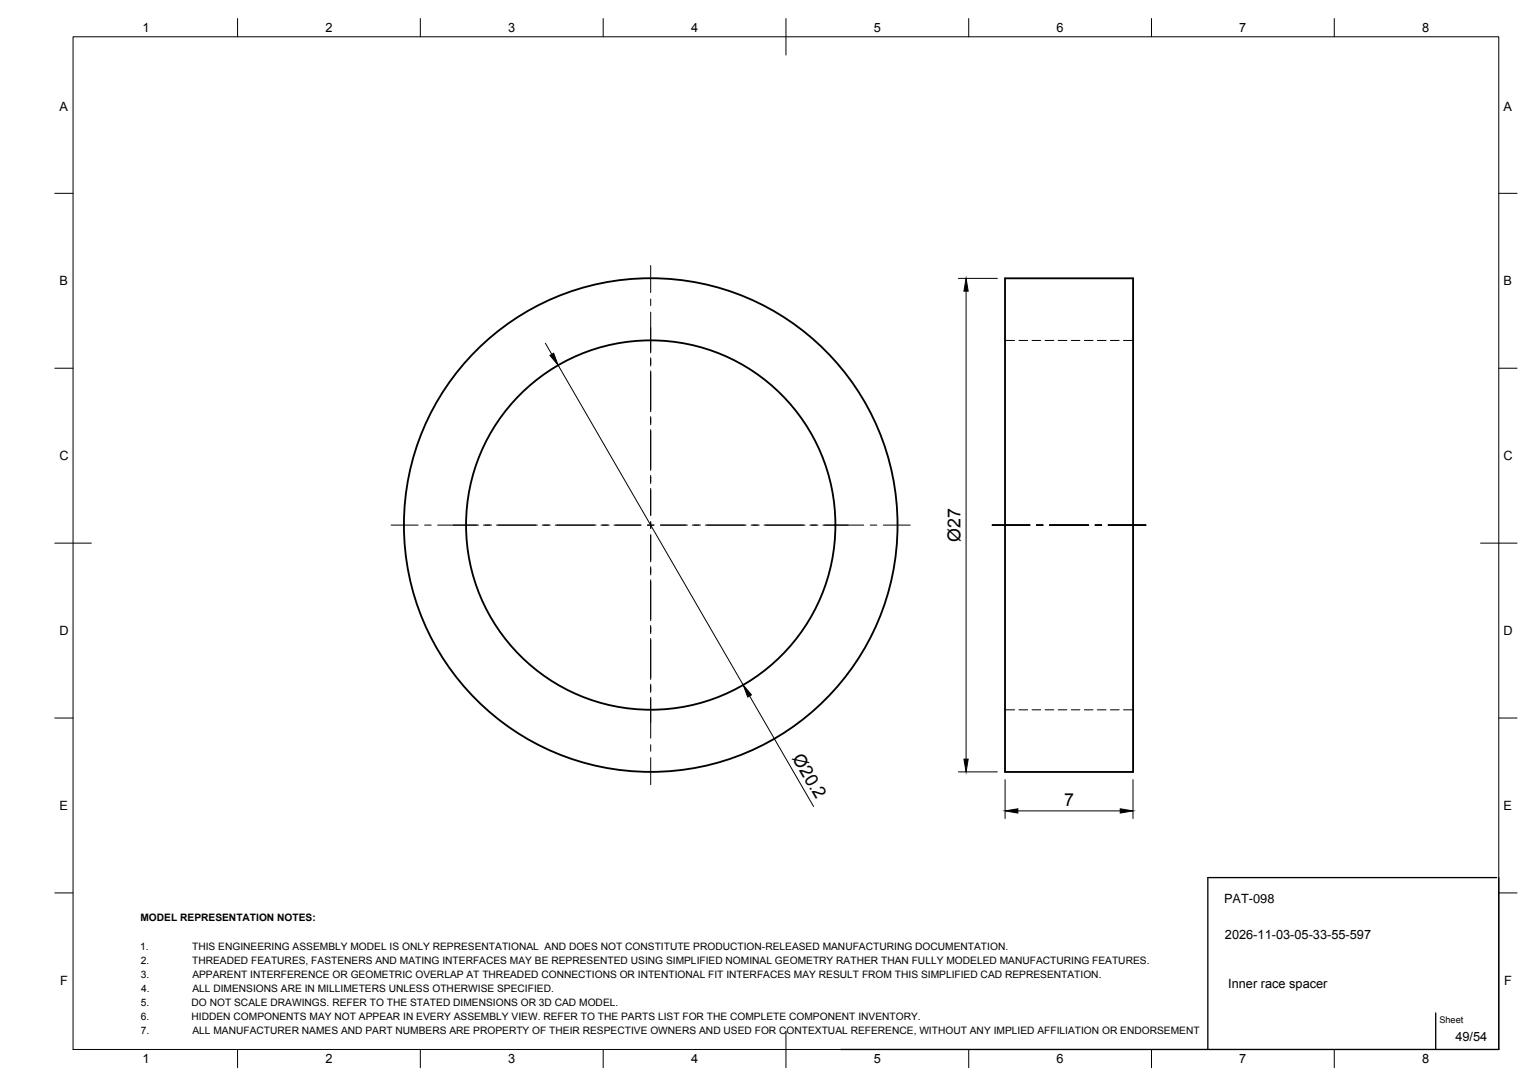
ISO-10303-21;
HEADER;
/* Generated by software containing ST-Developer
 * from STEP Tools, Inc. (www.steptools.com) 
 */

FILE_DESCRIPTION(
/* description */ ('Spring compression tester'),
/* implementation_level */ '2;1');

FILE_NAME(
/* name */ 'Inner race spacer.step',
/* time_stamp */ '2026-10-28T03:24:11-07:00',
/* author */ (''),
/* organization */ (''),
/* preprocessor_version */ 'ST-DEVELOPER v20.2',
/* originating_system */ 'Autodesk Translation Framework v15.17.0.0',
/* authorisation */ '');

FILE_SCHEMA (('AUTOMOTIVE_DESIGN { 1 0 10303 214 3 1 1 }'));
ENDSEC;

DATA;
#10=MECHANICAL_DESIGN_GEOMETRIC_PRESENTATION_REPRESENTATION('',(#1170),#43521);
#1035=SHAPE_REPRESENTATION_RELATIONSHIP('SRR','None',#43852,#1095);
#1095=ADVANCED_BREP_SHAPE_REPRESENTATION('',(#1239),#43512);
#1170=STYLED_ITEM('',(#44202),#1239);
#1239=MANIFOLD_SOLID_BREP('Body1',#18613);
#1569=FACE_BOUND('',#4514,.T.);
#1570=FACE_BOUND('',#4516,.T.);
#2120=PLANE('',#21061);
#2121=PLANE('',#21062);
#3142=FACE_OUTER_BOUND('',#4511,.T.);
#3143=FACE_OUTER_BOUND('',#4512,.T.);
#3144=FACE_OUTER_BOUND('',#4513,.T.);
#3145=FACE_OUTER_BOUND('',#4515,.T.);
#4511=EDGE_LOOP('',(#16795,#16796,#16797,#16798));
#4512=EDGE_LOOP('',(#16799,#16800,#16801,#16802));
#4513=EDGE_LOOP('',(#16803));
#4514=EDGE_LOOP('',(#16804));
#4515=EDGE_LOOP('',(#16805));
#4516=EDGE_LOOP('',(#16806));
#5937=LINE('',#42922,#7369);
#5938=LINE('',#42928,#7370);
#7369=VECTOR('',#26073,1.01);
#7370=VECTOR('',#26080,1.35);
#8092=CIRCLE('',#21056,1.01);
#8093=CIRCLE('',#21057,1.01);
#8094=CIRCLE('',#21059,1.35);
#8095=CIRCLE('',#21060,1.35);
#9671=VERTEX_POINT('',#42919);
#9672=VERTEX_POINT('',#42921);
#9673=VERTEX_POINT('',#42925);
#9674=VERTEX_POINT('',#42927);
#12062=EDGE_CURVE('',#9671,#9671,#8092,.T.);
#12063=EDGE_CURVE('',#9671,#9672,#5937,.T.);
#12064=EDGE_CURVE('',#9672,#9672,#8093,.T.);
#12065=EDGE_CURVE('',#9673,#9673,#8094,.T.);
#12066=EDGE_CURVE('',#9673,#9674,#5938,.T.);
#12067=EDGE_CURVE('',#9674,#9674,#8095,.T.);
#16795=ORIENTED_EDGE('',*,*,#12062,.F.);
#16796=ORIENTED_EDGE('',*,*,#12063,.T.);
#16797=ORIENTED_EDGE('',*,*,#12064,.T.);
#16798=ORIENTED_EDGE('',*,*,#12063,.F.);
#16799=ORIENTED_EDGE('',*,*,#12065,.F.);
#16800=ORIENTED_EDGE('',*,*,#12066,.T.);
#16801=ORIENTED_EDGE('',*,*,#12067,.T.);
#16802=ORIENTED_EDGE('',*,*,#12066,.F.);
#16803=ORIENTED_EDGE('',*,*,#12065,.T.);
#16804=ORIENTED_EDGE('',*,*,#12062,.T.);
#16805=ORIENTED_EDGE('',*,*,#12067,.F.);
#16806=ORIENTED_EDGE('',*,*,#12064,.F.);
#17475=CYLINDRICAL_SURFACE('',#21055,1.01);
#17476=CYLINDRICAL_SURFACE('',#21058,1.35);
#18466=ADVANCED_FACE('',(#3142),#17475,.F.);
#18467=ADVANCED_FACE('',(#3143),#17476,.T.);
#18468=ADVANCED_FACE('',(#3144,#1569),#2120,.T.);
#18469=ADVANCED_FACE('',(#3145,#1570),#2121,.F.);
#18613=CLOSED_SHELL('',(#18466,#18467,#18468,#18469));
#21054=AXIS2_PLACEMENT_3D('',#42917,#26067,#26068);
#21055=AXIS2_PLACEMENT_3D('',#42918,#26069,#26070);
#21056=AXIS2_PLACEMENT_3D('',#42920,#26071,#26072);
#21057=AXIS2_PLACEMENT_3D('',#42923,#26074,#26075);
#21058=AXIS2_PLACEMENT_3D('',#42924,#26076,#26077);
#21059=AXIS2_PLACEMENT_3D('',#42926,#26078,#26079);
#21060=AXIS2_PLACEMENT_3D('',#42929,#26081,#26082);
#21061=AXIS2_PLACEMENT_3D('',#42930,#26083,#26084);
#21062=AXIS2_PLACEMENT_3D('',#42931,#26085,#26086);
#26067=DIRECTION('axis',(0.,0.,1.));
#26068=DIRECTION('refdir',(1.,0.,0.));
#26069=DIRECTION('center_axis',(1.,0.,0.));
#26070=DIRECTION('ref_axis',(0.,0.,-1.));
#26071=DIRECTION('center_axis',(-1.,0.,0.));
#26072=DIRECTION('ref_axis',(0.,0.,-1.));
#26073=DIRECTION('',(-1.,0.,0.));
#26074=DIRECTION('center_axis',(-1.,0.,0.));
#26075=DIRECTION('ref_axis',(0.,0.,-1.));
#26076=DIRECTION('center_axis',(1.,0.,0.));
#26077=DIRECTION('ref_axis',(0.,0.,-1.));
#26078=DIRECTION('center_axis',(1.,0.,0.));
#26079=DIRECTION('ref_axis',(0.,0.,-1.));
#26080=DIRECTION('',(-1.,0.,0.));
#26081=DIRECTION('center_axis',(1.,0.,0.));
#26082=DIRECTION('ref_axis',(0.,0.,-1.));
#26083=DIRECTION('center_axis',(1.,0.,0.));
#26084=DIRECTION('ref_axis',(0.,0.,-1.));
#26085=DIRECTION('center_axis',(1.,0.,0.));
#26086=DIRECTION('ref_axis',(0.,0.,-1.));
#42917=CARTESIAN_POINT('',(0.,0.,0.));
#42918=CARTESIAN_POINT('Origin',(24.7,0.,4.));
#42919=CARTESIAN_POINT('',(25.4,-1.23689326713883E-16,5.01));
#42920=CARTESIAN_POINT('Origin',(25.4,0.,4.));
#42921=CARTESIAN_POINT('',(24.7,-1.23689326713883E-16,5.01));
#42922=CARTESIAN_POINT('',(24.7,-1.23689326713883E-16,5.01));
#42923=CARTESIAN_POINT('Origin',(24.7,0.,4.));
#42924=CARTESIAN_POINT('Origin',(24.7,0.,4.));
#42925=CARTESIAN_POINT('',(25.4,-1.65327317884893E-16,5.35));
#42926=CARTESIAN_POINT('Origin',(25.4,0.,4.));
#42927=CARTESIAN_POINT('',(24.7,-1.65327317884893E-16,5.35));
#42928=CARTESIAN_POINT('',(24.7,-1.65327317884893E-16,5.35));
#42929=CARTESIAN_POINT('Origin',(24.7,0.,4.));
#42930=CARTESIAN_POINT('Origin',(25.4,0.,4.));
#42931=CARTESIAN_POINT('Origin',(24.7,0.,4.));
#43444=UNCERTAINTY_MEASURE_WITH_UNIT(LENGTH_MEASURE(0.001),#43522,
'DISTANCE_ACCURACY_VALUE',
'Maximum model space distance between geometric entities at asserted c
onnectivities');
#43453=UNCERTAINTY_MEASURE_WITH_UNIT(LENGTH_MEASURE(0.001),#43522,
'DISTANCE_ACCURACY_VALUE',
'Maximum model space distance between geometric entities at asserted c
onnectivities');
#43512=(
GEOMETRIC_REPRESENTATION_CONTEXT(3)
GLOBAL_UNCERTAINTY_ASSIGNED_CONTEXT((#43444))
GLOBAL_UNIT_ASSIGNED_CONTEXT((#43522,#43524,#43525))
REPRESENTATION_CONTEXT('','3D')
);
#43521=(
GEOMETRIC_REPRESENTATION_CONTEXT(3)
GLOBAL_UNCERTAINTY_ASSIGNED_CONTEXT((#43453))
GLOBAL_UNIT_ASSIGNED_CONTEXT((#43522,#43524,#43525))
REPRESENTATION_CONTEXT('','3D')
);
#43522=(
LENGTH_UNIT()
NAMED_UNIT(*)
SI_UNIT(.CENTI.,.METRE.)
);
#43524=(
NAMED_UNIT(*)
PLANE_ANGLE_UNIT()
SI_UNIT($,.RADIAN.)
);
#43525=(
NAMED_UNIT(*)
SI_UNIT($,.STERADIAN.)
SOLID_ANGLE_UNIT()
);
#43584=SHAPE_DEFINITION_REPRESENTATION(#43771,#43852);
#43771=PRODUCT_DEFINITION_SHAPE('',$,#43920);
#43852=SHAPE_REPRESENTATION('',(#21054),#43512);
#43861=PRODUCT_DEFINITION_CONTEXT('part definition',#44064,'design');
#43920=PRODUCT_DEFINITION('Inner race spacer','Inner race spacer',#43987,
#43861);
#43987=PRODUCT_DEFINITION_FORMATION('',$,#44124);
#44064=APPLICATION_CONTEXT(
'Core Data for Automotive Mechanical Design Process');
#44065=PRODUCT_CONTEXT('part definition',#44064,'mechanical');
#44124=PRODUCT('Inner race spacer','Inner race spacer',
'Inner race spacer',(#44065));
#44196=COLOUR_RGB('Grey',0.48,0.52,0.57);
#44197=FILL_AREA_STYLE_COLOUR('',#44196);
#44198=FILL_AREA_STYLE('',(#44197));
#44199=SURFACE_STYLE_FILL_AREA(#44198);
#44200=SURFACE_SIDE_STYLE('',(#44199));
#44201=SURFACE_STYLE_USAGE(.BOTH.,#44200);
#44202=PRESENTATION_STYLE_ASSIGNMENT((#44201));
ENDSEC;
END-ISO-10303-21;
